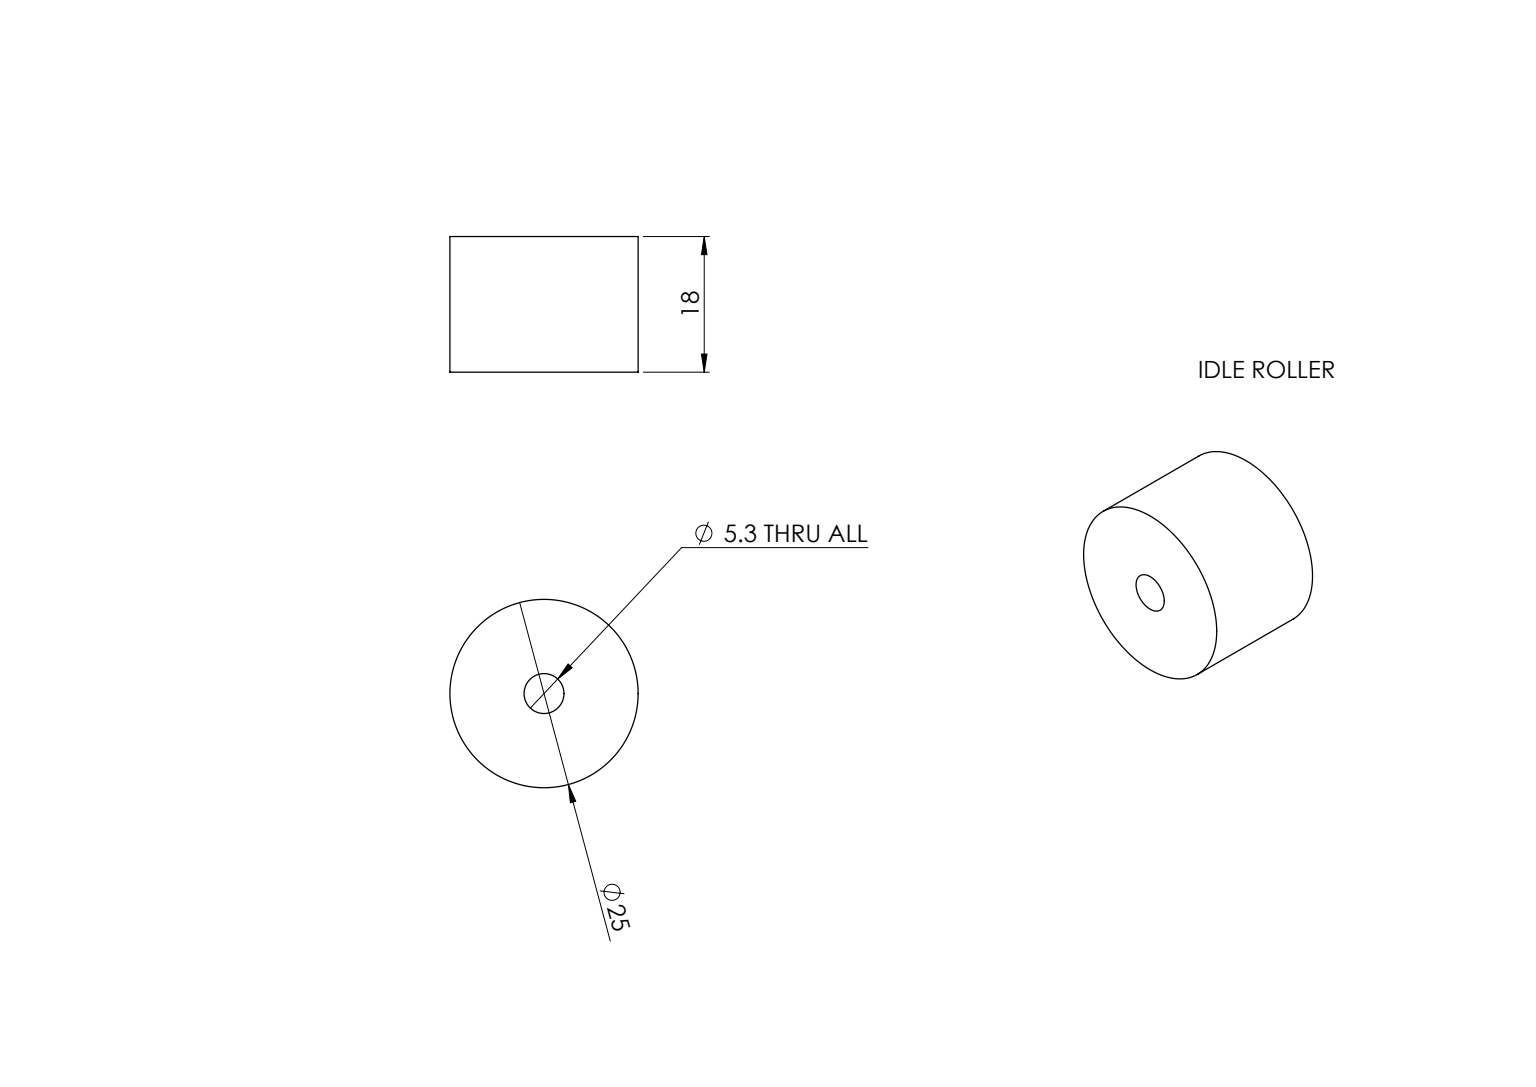
ISO-10303-21;
HEADER;
FILE_DESCRIPTION (('STEP AP214'),
    '1' );
FILE_NAME ('idle roller.step',
    '2026-10-25T07:12:54',
    ( '' ),
    ( '' ),
    'SwSTEP 2.0',
    'SolidWorks 2026',
    '' );
FILE_SCHEMA (( 'AUTOMOTIVE_DESIGN' ));
ENDSEC;

DATA;
#40=EDGE_CURVE ( 'NONE', #11408, #11811, #8258, .T. ) ;
#95=CIRCLE ( 'NONE', #11121, 2.649999999999988365 ) ;
#186=FACE_OUTER_BOUND ( 'NONE', #2806, .T. ) ;
#192=ADVANCED_FACE ( 'NONE', ( #1373 ), #9888, .F. ) ;
#252=FACE_BOUND ( 'NONE', #2068, .T. ) ;
#290=DIRECTION ( 'NONE',  ( 1.000000000000000000, 0.000000000000000000, 0.000000000000000000 ) ) ;
#352=CARTESIAN_POINT ( 'NONE',  ( -12.50000000000000000, 15.00000000000001599, 9.000000000000000000 ) ) ;
#363=ORIENTED_EDGE ( 'NONE', *, *, #770, .T. ) ;
#430=AXIS2_PLACEMENT_3D ( 'NONE', #5828, #10990, #3471 ) ;
#462=AXIS2_PLACEMENT_3D ( 'NONE', #7697, #5493, #290 ) ;
#488=EDGE_CURVE ( 'NONE', #4812, #10387, #3886, .T. ) ;
#550=EDGE_LOOP ( 'NONE', ( #6090, #11710, #2732, #9938 ) ) ;
#601=( NAMED_UNIT ( * ) SI_UNIT ( $, .STERADIAN. ) SOLID_ANGLE_UNIT ( ) );
#638=AXIS2_PLACEMENT_3D ( 'NONE', #4966, #12214, #3848 ) ;
#770=EDGE_CURVE ( 'NONE', #11811, #6957, #8397, .T. ) ;
#912=CYLINDRICAL_SURFACE ( 'NONE', #2246, 12.50000000000000000 ) ;
#979=FACE_OUTER_BOUND ( 'NONE', #5997, .T. ) ;
#1021=EDGE_CURVE ( 'NONE', #11408, #1099, #7809, .T. ) ;
#1087=MECHANICAL_DESIGN_GEOMETRIC_PRESENTATION_REPRESENTATION('',(#1966),#2431);
#1099=VERTEX_POINT ( 'NONE', #352 ) ;
#1123=DIRECTION ( 'NONE',  ( -0.000000000000000000, -0.000000000000000000, 1.000000000000000000 ) ) ;
#1148=APPLICATION_CONTEXT ( 'automotive_design' ) ;
#1211=VERTEX_POINT ( 'NONE', #1724 ) ;
#1341=PRESENTATION_STYLE_ASSIGNMENT (( #11485 ) ) ;
#1350=MECHANICAL_DESIGN_GEOMETRIC_PRESENTATION_REPRESENTATION('',(#8874),#12185);
#1373=FACE_OUTER_BOUND ( 'NONE', #11761, .T. ) ;
#1411=SHAPE_REPRESENTATION_RELATIONSHIP ( 'NONE' , 'NONE' ,  #8584, #2368 ) ;
#1588=( LENGTH_UNIT ( ) NAMED_UNIT ( * ) SI_UNIT ( .MILLI., .METRE. ) );
#1710=ADVANCED_FACE ( 'NONE', ( #1919 ), #4982, .T. ) ;
#1724=CARTESIAN_POINT ( 'NONE',  ( -2.649999999999988365, 15.00000000000001599, 9.000000000000000000 ) ) ;
#1733=AXIS2_PLACEMENT_3D ( 'NONE', #7089, #9091, #7918 ) ;
#1793=ADVANCED_FACE ( 'NONE', ( #252, #186 ), #7462, .F. ) ;
#1812=VECTOR ( 'NONE', #9209, 1000.000000000000000 ) ;
#1831=AXIS2_PLACEMENT_3D ( 'NONE', #5105, #11240, #6149 ) ;
#1919=FACE_OUTER_BOUND ( 'NONE', #11842, .T. ) ;
#1966=STYLED_ITEM ( 'NONE', ( #1341 ), #2368 ) ;
#2068=EDGE_LOOP ( 'NONE', ( #13556, #11987 ) ) ;
#2124=APPLICATION_CONTEXT ( 'automotive_design' ) ;
#2145=ORIENTED_EDGE ( 'NONE', *, *, #10169, .F. ) ;
#2189=CARTESIAN_POINT ( 'NONE',  ( 1.925929944387235853E-31, 15.00000000000001599, -9.000000000000000000 ) ) ;
#2215=CARTESIAN_POINT ( 'NONE',  ( 1.925929944387235853E-31, 15.00000000000001599, 15.00000000000000000 ) ) ;
#2246=AXIS2_PLACEMENT_3D ( 'NONE', #4313, #5295, #10464 ) ;
#2368=ADVANCED_BREP_SHAPE_REPRESENTATION ( '', ( #5429, #430 ), #11038 ) ;
#2431=( GEOMETRIC_REPRESENTATION_CONTEXT ( 3 ) GLOBAL_UNCERTAINTY_ASSIGNED_CONTEXT ( ( #3299 ) ) GLOBAL_UNIT_ASSIGNED_CONTEXT ( ( #3506, #4545, #13541 ) ) REPRESENTATION_CONTEXT ( 'NONE', 'WORKASPACE' ) );
#2708=CARTESIAN_POINT ( 'NONE',  ( 2.649999999999988365, 15.00000000000001599, 15.00000000000000000 ) ) ;
#2724=CARTESIAN_POINT ( 'NONE',  ( 2.649999999999989697, 15.00000000000001599, -9.000000000000001776 ) ) ;
#2726=FACE_OUTER_BOUND ( 'NONE', #7147, .T. ) ;
#2732=ORIENTED_EDGE ( 'NONE', *, *, #3011, .T. ) ;
#2806=EDGE_LOOP ( 'NONE', ( #2145, #12723 ) ) ;
#3011=EDGE_CURVE ( 'NONE', #4812, #8256, #8875, .T. ) ;
#3032=CARTESIAN_POINT ( 'NONE',  ( 1.925929944387235853E-31, 15.00000000000001599, 9.000000000000000000 ) ) ;
#3299=UNCERTAINTY_MEASURE_WITH_UNIT (LENGTH_MEASURE( 1.000000000000000082E-05 ), #3506, 'distance_accuracy_value', 'NONE');
#3306=DIRECTION ( 'NONE',  ( 1.000000000000000000, 0.000000000000000000, -0.000000000000000000 ) ) ;
#3397=ORIENTED_EDGE ( 'NONE', *, *, #10169, .T. ) ;
#3410=CYLINDRICAL_SURFACE ( 'NONE', #462, 2.649999999999988365 ) ;
#3429=LINE ( 'NONE', #7652, #12341 ) ;
#3464=PRODUCT ( 'idle roller', 'idle roller', '', ( #13419 ) ) ;
#3471=DIRECTION ( 'NONE',  ( 1.000000000000000000, 0.000000000000000000, 0.000000000000000000 ) ) ;
#3490=CIRCLE ( 'NONE', #5926, 12.50000000000000000 ) ;
#3506=( LENGTH_UNIT ( ) NAMED_UNIT ( * ) SI_UNIT ( .MILLI., .METRE. ) );
#3848=DIRECTION ( 'NONE',  ( 1.000000000000000000, 0.000000000000000000, 0.000000000000000000 ) ) ;
#3878=CARTESIAN_POINT ( 'NONE',  ( -2.649999999999988365, 15.00000000000001599, 15.00000000000000000 ) ) ;
#3886=CIRCLE ( 'NONE', #12276, 2.649999999999989697 ) ;
#4017=( NAMED_UNIT ( * ) PLANE_ANGLE_UNIT ( ) SI_UNIT ( $, .RADIAN. ) );
#4074=CIRCLE ( 'NONE', #6086, 2.649999999999988365 ) ;
#4180=EDGE_CURVE ( 'NONE', #1211, #8256, #4074, .T. ) ;
#4220=CARTESIAN_POINT ( 'NONE',  ( 12.50000000000000000, 15.00000000000001776, -9.000000000000000000 ) ) ;
#4313=CARTESIAN_POINT ( 'NONE',  ( 1.925929944387235853E-31, 15.00000000000001599, 9.000000000000000000 ) ) ;
#4367=DIRECTION ( 'NONE',  ( -0.000000000000000000, -0.000000000000000000, 1.000000000000000000 ) ) ;
#4438=CARTESIAN_POINT ( 'NONE',  ( 2.649999999999988365, 15.00000000000001599, 9.000000000000000000 ) ) ;
#4476=DIRECTION ( 'NONE',  ( 0.000000000000000000, 0.000000000000000000, 1.000000000000000000 ) ) ;
#4539=UNCERTAINTY_MEASURE_WITH_UNIT (LENGTH_MEASURE( 1.000000000000000082E-05 ), #10304, 'distance_accuracy_value', 'NONE');
#4545=( NAMED_UNIT ( * ) PLANE_ANGLE_UNIT ( ) SI_UNIT ( $, .RADIAN. ) );
#4676=ORIENTED_EDGE ( 'NONE', *, *, #1021, .F. ) ;
#4752=CARTESIAN_POINT ( 'NONE',  ( -12.50000000000000000, 15.00000000000001599, -9.000000000000000000 ) ) ;
#4812=VERTEX_POINT ( 'NONE', #2724 ) ;
#4940=CLOSED_SHELL ( 'NONE', ( #192, #5048, #1710, #6216, #1793, #5265 ) ) ;
#4966=CARTESIAN_POINT ( 'NONE',  ( 1.925929944387235853E-31, 15.00000000000001599, 9.000000000000000000 ) ) ;
#4982=CYLINDRICAL_SURFACE ( 'NONE', #5847, 12.50000000000000000 ) ;
#5048=ADVANCED_FACE ( 'NONE', ( #979 ), #912, .T. ) ;
#5063=FILL_AREA_STYLE_COLOUR ( '', #5104 ) ;
#5104=COLOUR_RGB ( '',0.8941176470588234615, 0.8941176470588234615, 0.8941176470588234615 ) ;
#5105=CARTESIAN_POINT ( 'NONE',  ( 1.925929944387235853E-31, 15.00000000000001599, 9.000000000000000000 ) ) ;
#5157=CARTESIAN_POINT ( 'NONE',  ( 1.925929944387235853E-31, 15.00000000000001599, 9.000000000000000000 ) ) ;
#5163=AXIS2_PLACEMENT_3D ( 'NONE', #2215, #4367, #5549 ) ;
#5265=ADVANCED_FACE ( 'NONE', ( #12866 ), #3410, .F. ) ;
#5287=DIRECTION ( 'NONE',  ( 0.000000000000000000, 0.000000000000000000, 1.000000000000000000 ) ) ;
#5295=DIRECTION ( 'NONE',  ( -0.000000000000000000, -0.000000000000000000, -1.000000000000000000 ) ) ;
#5388=ORIENTED_EDGE ( 'NONE', *, *, #3011, .F. ) ;
#5429=MANIFOLD_SOLID_BREP ( 'M5 Clearance Hole1', #4940 ) ;
#5458=ORIENTED_EDGE ( 'NONE', *, *, #6601, .T. ) ;
#5493=DIRECTION ( 'NONE',  ( -0.000000000000000000, -0.000000000000000000, 1.000000000000000000 ) ) ;
#5549=DIRECTION ( 'NONE',  ( 1.000000000000000000, 0.000000000000000000, 0.000000000000000000 ) ) ;
#5828=CARTESIAN_POINT ( 'NONE',  ( 0.000000000000000000, 0.000000000000000000, 0.000000000000000000 ) ) ;
#5847=AXIS2_PLACEMENT_3D ( 'NONE', #3032, #7259, #7333 ) ;
#5926=AXIS2_PLACEMENT_3D ( 'NONE', #11504, #5287, #10391 ) ;
#5992=PLANE ( 'NONE',  #1733 ) ;
#5997=EDGE_LOOP ( 'NONE', ( #4676, #7269, #363, #8275 ) ) ;
#6086=AXIS2_PLACEMENT_3D ( 'NONE', #7237, #8408, #9303 ) ;
#6090=ORIENTED_EDGE ( 'NONE', *, *, #6601, .F. ) ;
#6140=EDGE_CURVE ( 'NONE', #1099, #6957, #3429, .T. ) ;
#6149=DIRECTION ( 'NONE',  ( 1.000000000000000000, 0.000000000000000000, 0.000000000000000000 ) ) ;
#6216=ADVANCED_FACE ( 'NONE', ( #12130, #2726 ), #5992, .T. ) ;
#6601=EDGE_CURVE ( 'NONE', #10387, #1211, #11345, .T. ) ;
#6841=PRODUCT_DEFINITION_FORMATION_WITH_SPECIFIED_SOURCE ( 'ANY', '', #3464, .NOT_KNOWN. ) ;
#6957=VERTEX_POINT ( 'NONE', #4752 ) ;
#7089=CARTESIAN_POINT ( 'NONE',  ( 1.925929944387235853E-31, 15.00000000000001599, 9.000000000000000000 ) ) ;
#7147=EDGE_LOOP ( 'NONE', ( #9149, #8825 ) ) ;
#7228=SHAPE_DEFINITION_REPRESENTATION ( #11846, #8584 ) ;
#7237=CARTESIAN_POINT ( 'NONE',  ( 1.925929944387235853E-31, 15.00000000000001599, 9.000000000000000000 ) ) ;
#7259=DIRECTION ( 'NONE',  ( -0.000000000000000000, -0.000000000000000000, -1.000000000000000000 ) ) ;
#7269=ORIENTED_EDGE ( 'NONE', *, *, #40, .T. ) ;
#7333=DIRECTION ( 'NONE',  ( -1.000000000000000000, 0.000000000000000000, 0.000000000000000000 ) ) ;
#7380=CARTESIAN_POINT ( 'NONE',  ( 1.925929944387235853E-31, 15.00000000000001599, -9.000000000000001776 ) ) ;
#7462=PLANE ( 'NONE',  #9813 ) ;
#7652=CARTESIAN_POINT ( 'NONE',  ( -12.50000000000000000, 15.00000000000001599, 9.000000000000000000 ) ) ;
#7697=CARTESIAN_POINT ( 'NONE',  ( 1.925929944387235853E-31, 15.00000000000001599, 15.00000000000000000 ) ) ;
#7777=CARTESIAN_POINT ( 'NONE',  ( 12.50000000000000000, 15.00000000000001776, 9.000000000000000000 ) ) ;
#7809=CIRCLE ( 'NONE', #1831, 12.50000000000000000 ) ;
#7918=DIRECTION ( 'NONE',  ( 1.000000000000000000, 0.000000000000000000, -0.000000000000000000 ) ) ;
#8080=ORIENTED_EDGE ( 'NONE', *, *, #9814, .F. ) ;
#8243=FILL_AREA_STYLE ('',( #5063 ) ) ;
#8256=VERTEX_POINT ( 'NONE', #4438 ) ;
#8258=LINE ( 'NONE', #12530, #11097 ) ;
#8274=DIRECTION ( 'NONE',  ( -0.000000000000000000, -0.000000000000000000, 1.000000000000000000 ) ) ;
#8275=ORIENTED_EDGE ( 'NONE', *, *, #6140, .F. ) ;
#8397=CIRCLE ( 'NONE', #11914, 12.50000000000000000 ) ;
#8408=DIRECTION ( 'NONE',  ( 0.000000000000000000, 0.000000000000000000, 1.000000000000000000 ) ) ;
#8584=SHAPE_REPRESENTATION ( 'idle roller', ( #430 ), #11038 ) ;
#8825=ORIENTED_EDGE ( 'NONE', *, *, #1021, .T. ) ;
#8874=STYLED_ITEM('',(#13691),#5429);
#8875=LINE ( 'NONE', #2708, #10656 ) ;
#8947=CARTESIAN_POINT ( 'NONE',  ( 1.925929944387235853E-31, 15.00000000000001599, -9.000000000000000000 ) ) ;
#9008=DIRECTION ( 'NONE',  ( 0.000000000000000000, 0.000000000000000000, 1.000000000000000000 ) ) ;
#9054=CIRCLE ( 'NONE', #638, 12.50000000000000000 ) ;
#9091=DIRECTION ( 'NONE',  ( 0.000000000000000000, 0.000000000000000000, 1.000000000000000000 ) ) ;
#9149=ORIENTED_EDGE ( 'NONE', *, *, #9814, .T. ) ;
#9208=CARTESIAN_POINT ( 'NONE',  ( -2.649999999999989697, 15.00000000000001599, -9.000000000000001776 ) ) ;
#9209=DIRECTION ( 'NONE',  ( -0.000000000000000000, -0.000000000000000000, 1.000000000000000000 ) ) ;
#9303=DIRECTION ( 'NONE',  ( 1.000000000000000000, 0.000000000000000000, 0.000000000000000000 ) ) ;
#9363=DIRECTION ( 'NONE',  ( 0.000000000000000000, 0.000000000000000000, 1.000000000000000000 ) ) ;
#9813=AXIS2_PLACEMENT_3D ( 'NONE', #2189, #4476, #3306 ) ;
#9814=EDGE_CURVE ( 'NONE', #1099, #11408, #9054, .T. ) ;
#9888=CYLINDRICAL_SURFACE ( 'NONE', #5163, 2.649999999999988365 ) ;
#9938=ORIENTED_EDGE ( 'NONE', *, *, #13384, .T. ) ;
#10034=DIRECTION ( 'NONE',  ( -0.000000000000000000, -0.000000000000000000, 1.000000000000000000 ) ) ;
#10036=PRODUCT_DEFINITION ( 'UNKNOWN', '', #6841, #11358 ) ;
#10052=ORIENTED_EDGE ( 'NONE', *, *, #40, .F. ) ;
#10169=EDGE_CURVE ( 'NONE', #6957, #11811, #3490, .T. ) ;
#10304=( LENGTH_UNIT ( ) NAMED_UNIT ( * ) SI_UNIT ( .MILLI., .METRE. ) );
#10387=VERTEX_POINT ( 'NONE', #9208 ) ;
#10391=DIRECTION ( 'NONE',  ( 1.000000000000000000, 0.000000000000000000, 0.000000000000000000 ) ) ;
#10464=DIRECTION ( 'NONE',  ( -1.000000000000000000, 0.000000000000000000, 0.000000000000000000 ) ) ;
#10503=( NAMED_UNIT ( * ) PLANE_ANGLE_UNIT ( ) SI_UNIT ( $, .RADIAN. ) );
#10610=CARTESIAN_POINT ( 'NONE',  ( 1.925929944387235853E-31, 15.00000000000001599, -9.000000000000001776 ) ) ;
#10656=VECTOR ( 'NONE', #10034, 1000.000000000000000 ) ;
#10688=AXIS2_PLACEMENT_3D ( 'NONE', #7380, #1123, #11650 ) ;
#10895=CIRCLE ( 'NONE', #10688, 2.649999999999989697 ) ;
#10951=DIRECTION ( 'NONE',  ( -0.000000000000000000, -0.000000000000000000, -1.000000000000000000 ) ) ;
#10990=DIRECTION ( 'NONE',  ( 0.000000000000000000, 0.000000000000000000, 1.000000000000000000 ) ) ;
#11038=( GEOMETRIC_REPRESENTATION_CONTEXT ( 3 ) GLOBAL_UNCERTAINTY_ASSIGNED_CONTEXT ( ( #4539 ) ) GLOBAL_UNIT_ASSIGNED_CONTEXT ( ( #10304, #4017, #601 ) ) REPRESENTATION_CONTEXT ( 'NONE', 'WORKASPACE' ) );
#11097=VECTOR ( 'NONE', #11424, 1000.000000000000000 ) ;
#11121=AXIS2_PLACEMENT_3D ( 'NONE', #5157, #9363, #11149 ) ;
#11149=DIRECTION ( 'NONE',  ( 1.000000000000000000, 0.000000000000000000, 0.000000000000000000 ) ) ;
#11211=ORIENTED_EDGE ( 'NONE', *, *, #4180, .F. ) ;
#11240=DIRECTION ( 'NONE',  ( 0.000000000000000000, 0.000000000000000000, 1.000000000000000000 ) ) ;
#11286=DIRECTION ( 'NONE',  ( 1.000000000000000000, 0.000000000000000000, 0.000000000000000000 ) ) ;
#11345=LINE ( 'NONE', #3878, #1812 ) ;
#11358=PRODUCT_DEFINITION_CONTEXT ( 'detailed design', #2124, 'design' ) ;
#11408=VERTEX_POINT ( 'NONE', #7777 ) ;
#11411=SURFACE_SIDE_STYLE ('',( #12442 ) ) ;
#11424=DIRECTION ( 'NONE',  ( -0.000000000000000000, -0.000000000000000000, -1.000000000000000000 ) ) ;
#11485=SURFACE_STYLE_USAGE ( .BOTH. , #11411 ) ;
#11504=CARTESIAN_POINT ( 'NONE',  ( 1.925929944387235853E-31, 15.00000000000001599, -9.000000000000000000 ) ) ;
#11520=DIRECTION ( 'NONE',  ( 1.000000000000000000, 0.000000000000000000, 0.000000000000000000 ) ) ;
#11551=( NAMED_UNIT ( * ) SI_UNIT ( $, .STERADIAN. ) SOLID_ANGLE_UNIT ( ) );
#11650=DIRECTION ( 'NONE',  ( 1.000000000000000000, 0.000000000000000000, 0.000000000000000000 ) ) ;
#11710=ORIENTED_EDGE ( 'NONE', *, *, #488, .F. ) ;
#11761=EDGE_LOOP ( 'NONE', ( #12270, #5458, #13222, #5388 ) ) ;
#11811=VERTEX_POINT ( 'NONE', #4220 ) ;
#11842=EDGE_LOOP ( 'NONE', ( #10052, #8080, #12069, #3397 ) ) ;
#11846=PRODUCT_DEFINITION_SHAPE ( 'NONE', 'NONE',  #10036 ) ;
#11914=AXIS2_PLACEMENT_3D ( 'NONE', #8947, #9008, #11286 ) ;
#11987=ORIENTED_EDGE ( 'NONE', *, *, #12929, .T. ) ;
#12069=ORIENTED_EDGE ( 'NONE', *, *, #6140, .T. ) ;
#12130=FACE_BOUND ( 'NONE', #13607, .T. ) ;
#12185=( GEOMETRIC_REPRESENTATION_CONTEXT ( 3 ) GLOBAL_UNCERTAINTY_ASSIGNED_CONTEXT ( ( #12457 ) ) GLOBAL_UNIT_ASSIGNED_CONTEXT ( ( #1588, #10503, #11551 ) ) REPRESENTATION_CONTEXT ( 'NONE', 'WORKASPACE' ) );
#12214=DIRECTION ( 'NONE',  ( 0.000000000000000000, 0.000000000000000000, 1.000000000000000000 ) ) ;
#12270=ORIENTED_EDGE ( 'NONE', *, *, #12929, .F. ) ;
#12276=AXIS2_PLACEMENT_3D ( 'NONE', #10610, #8274, #11520 ) ;
#12341=VECTOR ( 'NONE', #10951, 1000.000000000000000 ) ;
#12442=SURFACE_STYLE_FILL_AREA ( #8243 ) ;
#12457=UNCERTAINTY_MEASURE_WITH_UNIT (LENGTH_MEASURE( 1.000000000000000082E-05 ), #1588, 'distance_accuracy_value', 'NONE');
#12530=CARTESIAN_POINT ( 'NONE',  ( 12.50000000000000000, 15.00000000000001776, 9.000000000000000000 ) ) ;
#12723=ORIENTED_EDGE ( 'NONE', *, *, #770, .F. ) ;
#12866=FACE_OUTER_BOUND ( 'NONE', #550, .T. ) ;
#12891=ORIENTED_EDGE ( 'NONE', *, *, #13384, .F. ) ;
#12929=EDGE_CURVE ( 'NONE', #10387, #4812, #10895, .T. ) ;
#13222=ORIENTED_EDGE ( 'NONE', *, *, #4180, .T. ) ;
#13384=EDGE_CURVE ( 'NONE', #8256, #1211, #95, .T. ) ;
#13419=PRODUCT_CONTEXT ( 'NONE', #1148, 'mechanical' ) ;
#13541=( NAMED_UNIT ( * ) SI_UNIT ( $, .STERADIAN. ) SOLID_ANGLE_UNIT ( ) );
#13556=ORIENTED_EDGE ( 'NONE', *, *, #488, .T. ) ;
#13607=EDGE_LOOP ( 'NONE', ( #12891, #11211 ) ) ;
#13685=COLOUR_RGB('Light Blue',0.38,0.62,0.78);
#13686=FILL_AREA_STYLE_COLOUR('',#13685);
#13687=FILL_AREA_STYLE('',(#13686));
#13688=SURFACE_STYLE_FILL_AREA(#13687);
#13689=SURFACE_SIDE_STYLE('',(#13688));
#13690=SURFACE_STYLE_USAGE(.BOTH.,#13689);
#13691=PRESENTATION_STYLE_ASSIGNMENT((#13690));
ENDSEC;
END-ISO-10303-21;
